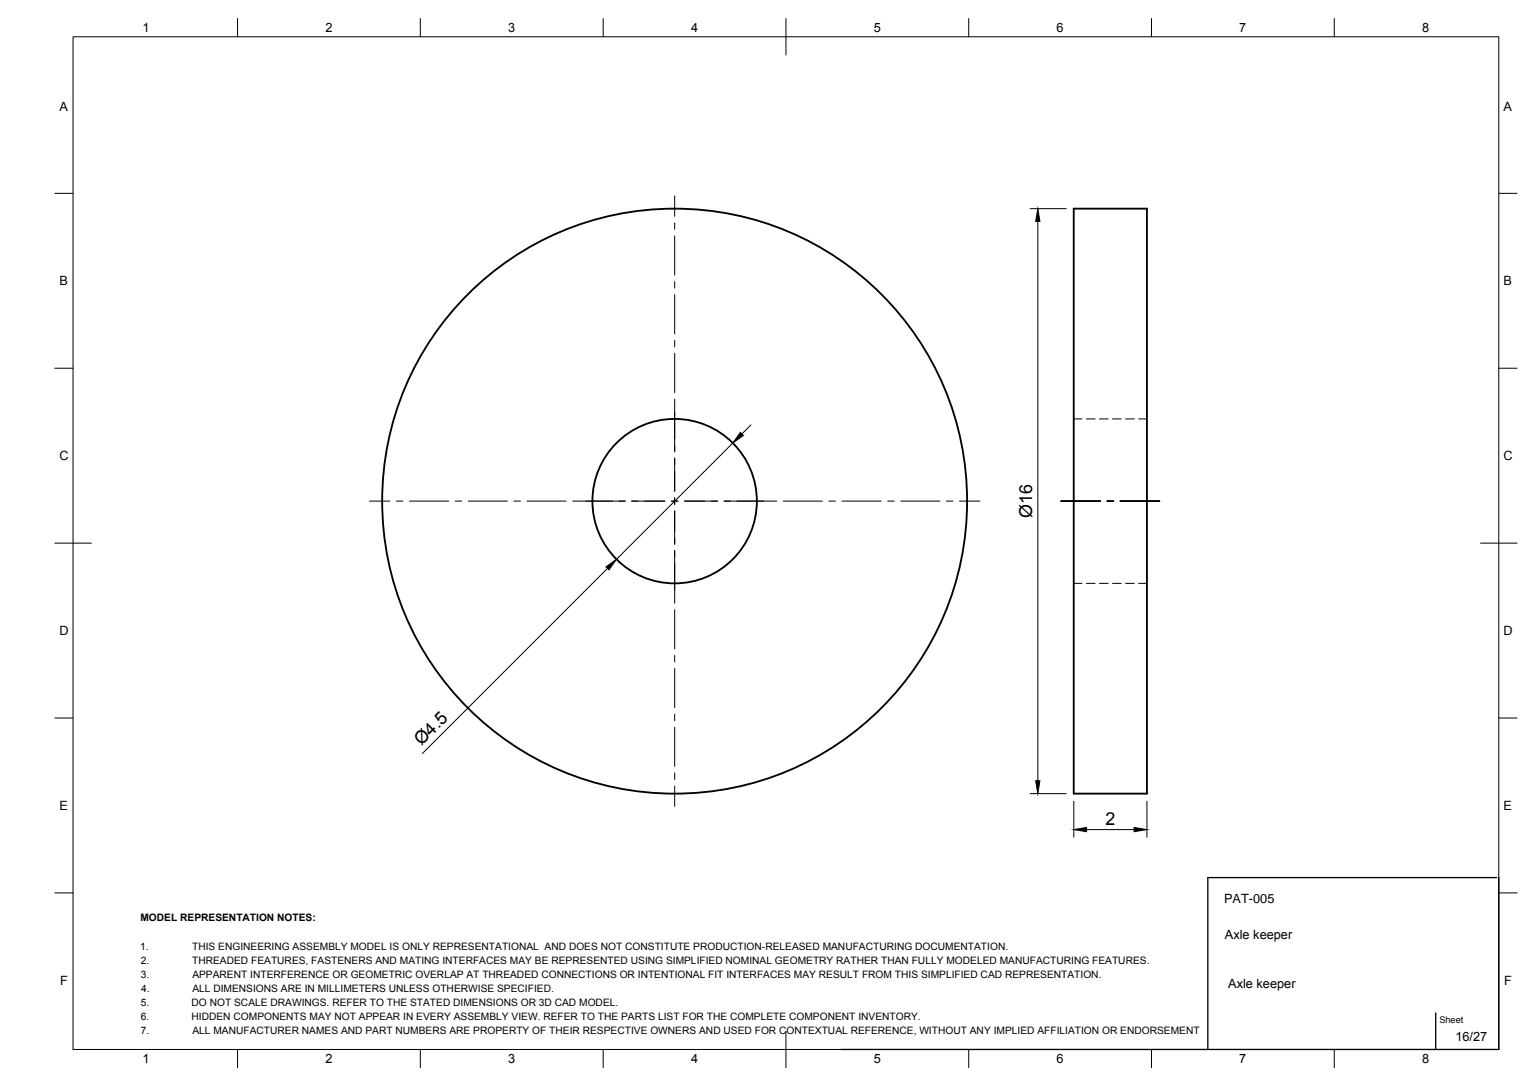
ISO-10303-21;
HEADER;
/* Generated by software containing ST-Developer
 * from STEP Tools, Inc. (www.steptools.com) 
 */

FILE_DESCRIPTION(
/* description */ ('Ball-race swivel caster'),
/* implementation_level */ '2;1');

FILE_NAME(
/* name */ 'Axle keeper.step',
/* time_stamp */ '2026-10-29T16:15:51-07:00',
/* author */ (''),
/* organization */ (''),
/* preprocessor_version */ 'ST-DEVELOPER v20.2',
/* originating_system */ 'Autodesk Translation Framework v15.17.0.0',
/* authorisation */ '');

FILE_SCHEMA (('AUTOMOTIVE_DESIGN { 1 0 10303 214 3 1 1 }'));
ENDSEC;

DATA;
#10=MECHANICAL_DESIGN_GEOMETRIC_PRESENTATION_REPRESENTATION('',(#318),#7816);
#269=SHAPE_REPRESENTATION_RELATIONSHIP('SRR','None',#7916,#289);
#289=ADVANCED_BREP_SHAPE_REPRESENTATION('',(#354),#7805);
#318=STYLED_ITEM('',(#8097),#354);
#354=MANIFOLD_SOLID_BREP('Body1',#3724);
#420=FACE_BOUND('',#916,.T.);
#421=FACE_BOUND('',#918,.T.);
#489=PLANE('',#4293);
#490=PLANE('',#4294);
#653=FACE_OUTER_BOUND('',#913,.T.);
#654=FACE_OUTER_BOUND('',#914,.T.);
#655=FACE_OUTER_BOUND('',#915,.T.);
#656=FACE_OUTER_BOUND('',#917,.T.);
#913=EDGE_LOOP('',(#3121,#3122,#3123,#3124));
#914=EDGE_LOOP('',(#3125,#3126,#3127,#3128));
#915=EDGE_LOOP('',(#3129));
#916=EDGE_LOOP('',(#3130));
#917=EDGE_LOOP('',(#3131));
#918=EDGE_LOOP('',(#3132));
#1119=LINE('',#7101,#1274);
#1120=LINE('',#7107,#1275);
#1274=VECTOR('',#5251,0.225);
#1275=VECTOR('',#5258,0.8);
#1493=CIRCLE('',#4288,0.225);
#1494=CIRCLE('',#4289,0.225);
#1495=CIRCLE('',#4291,0.8);
#1496=CIRCLE('',#4292,0.8);
#1827=VERTEX_POINT('',#7098);
#1828=VERTEX_POINT('',#7100);
#1829=VERTEX_POINT('',#7104);
#1830=VERTEX_POINT('',#7106);
#2280=EDGE_CURVE('',#1827,#1827,#1493,.T.);
#2281=EDGE_CURVE('',#1827,#1828,#1119,.T.);
#2282=EDGE_CURVE('',#1828,#1828,#1494,.T.);
#2283=EDGE_CURVE('',#1829,#1829,#1495,.T.);
#2284=EDGE_CURVE('',#1829,#1830,#1120,.T.);
#2285=EDGE_CURVE('',#1830,#1830,#1496,.T.);
#3121=ORIENTED_EDGE('',*,*,#2280,.F.);
#3122=ORIENTED_EDGE('',*,*,#2281,.T.);
#3123=ORIENTED_EDGE('',*,*,#2282,.T.);
#3124=ORIENTED_EDGE('',*,*,#2281,.F.);
#3125=ORIENTED_EDGE('',*,*,#2283,.F.);
#3126=ORIENTED_EDGE('',*,*,#2284,.T.);
#3127=ORIENTED_EDGE('',*,*,#2285,.T.);
#3128=ORIENTED_EDGE('',*,*,#2284,.F.);
#3129=ORIENTED_EDGE('',*,*,#2283,.T.);
#3130=ORIENTED_EDGE('',*,*,#2280,.T.);
#3131=ORIENTED_EDGE('',*,*,#2285,.F.);
#3132=ORIENTED_EDGE('',*,*,#2282,.F.);
#3473=CYLINDRICAL_SURFACE('',#4287,0.225);
#3474=CYLINDRICAL_SURFACE('',#4290,0.8);
#3624=ADVANCED_FACE('',(#653),#3473,.F.);
#3625=ADVANCED_FACE('',(#654),#3474,.T.);
#3626=ADVANCED_FACE('',(#655,#420),#489,.T.);
#3627=ADVANCED_FACE('',(#656,#421),#490,.F.);
#3724=CLOSED_SHELL('',(#3624,#3625,#3626,#3627));
#4286=AXIS2_PLACEMENT_3D('',#7096,#5245,#5246);
#4287=AXIS2_PLACEMENT_3D('',#7097,#5247,#5248);
#4288=AXIS2_PLACEMENT_3D('',#7099,#5249,#5250);
#4289=AXIS2_PLACEMENT_3D('',#7102,#5252,#5253);
#4290=AXIS2_PLACEMENT_3D('',#7103,#5254,#5255);
#4291=AXIS2_PLACEMENT_3D('',#7105,#5256,#5257);
#4292=AXIS2_PLACEMENT_3D('',#7108,#5259,#5260);
#4293=AXIS2_PLACEMENT_3D('',#7109,#5261,#5262);
#4294=AXIS2_PLACEMENT_3D('',#7110,#5263,#5264);
#5245=DIRECTION('axis',(0.,0.,1.));
#5246=DIRECTION('refdir',(1.,0.,0.));
#5247=DIRECTION('center_axis',(0.,1.,0.));
#5248=DIRECTION('ref_axis',(1.,0.,0.));
#5249=DIRECTION('center_axis',(0.,-1.,0.));
#5250=DIRECTION('ref_axis',(1.,0.,0.));
#5251=DIRECTION('',(0.,-1.,0.));
#5252=DIRECTION('center_axis',(0.,-1.,0.));
#5253=DIRECTION('ref_axis',(1.,0.,0.));
#5254=DIRECTION('center_axis',(0.,1.,0.));
#5255=DIRECTION('ref_axis',(1.,0.,0.));
#5256=DIRECTION('center_axis',(0.,1.,0.));
#5257=DIRECTION('ref_axis',(1.,0.,0.));
#5258=DIRECTION('',(0.,-1.,0.));
#5259=DIRECTION('center_axis',(0.,1.,0.));
#5260=DIRECTION('ref_axis',(1.,0.,0.));
#5261=DIRECTION('center_axis',(0.,1.,0.));
#5262=DIRECTION('ref_axis',(1.,0.,0.));
#5263=DIRECTION('center_axis',(0.,1.,0.));
#5264=DIRECTION('ref_axis',(1.,0.,0.));
#7096=CARTESIAN_POINT('',(0.,0.,0.));
#7097=CARTESIAN_POINT('Origin',(0.,2.2,4.));
#7098=CARTESIAN_POINT('',(-0.225,2.4,4.));
#7099=CARTESIAN_POINT('Origin',(0.,2.4,4.));
#7100=CARTESIAN_POINT('',(-0.225,2.2,4.));
#7101=CARTESIAN_POINT('',(-0.225,2.2,4.));
#7102=CARTESIAN_POINT('Origin',(0.,2.2,4.));
#7103=CARTESIAN_POINT('Origin',(0.,2.2,4.));
#7104=CARTESIAN_POINT('',(-0.8,2.4,4.));
#7105=CARTESIAN_POINT('Origin',(0.,2.4,4.));
#7106=CARTESIAN_POINT('',(-0.8,2.2,4.));
#7107=CARTESIAN_POINT('',(-0.8,2.2,4.));
#7108=CARTESIAN_POINT('Origin',(0.,2.2,4.));
#7109=CARTESIAN_POINT('Origin',(0.,2.4,4.));
#7110=CARTESIAN_POINT('Origin',(0.,2.2,4.));
#7778=UNCERTAINTY_MEASURE_WITH_UNIT(LENGTH_MEASURE(0.001),#7817,
'DISTANCE_ACCURACY_VALUE',
'Maximum model space distance between geometric entities at asserted c
onnectivities');
#7789=UNCERTAINTY_MEASURE_WITH_UNIT(LENGTH_MEASURE(0.001),#7817,
'DISTANCE_ACCURACY_VALUE',
'Maximum model space distance between geometric entities at asserted c
onnectivities');
#7805=(
GEOMETRIC_REPRESENTATION_CONTEXT(3)
GLOBAL_UNCERTAINTY_ASSIGNED_CONTEXT((#7778))
GLOBAL_UNIT_ASSIGNED_CONTEXT((#7817,#7819,#7820))
REPRESENTATION_CONTEXT('','3D')
);
#7816=(
GEOMETRIC_REPRESENTATION_CONTEXT(3)
GLOBAL_UNCERTAINTY_ASSIGNED_CONTEXT((#7789))
GLOBAL_UNIT_ASSIGNED_CONTEXT((#7817,#7819,#7820))
REPRESENTATION_CONTEXT('','3D')
);
#7817=(
LENGTH_UNIT()
NAMED_UNIT(*)
SI_UNIT(.CENTI.,.METRE.)
);
#7819=(
NAMED_UNIT(*)
PLANE_ANGLE_UNIT()
SI_UNIT($,.RADIAN.)
);
#7820=(
NAMED_UNIT(*)
SI_UNIT($,.STERADIAN.)
SOLID_ANGLE_UNIT()
);
#7836=SHAPE_DEFINITION_REPRESENTATION(#7870,#7916);
#7870=PRODUCT_DEFINITION_SHAPE('',$,#7943);
#7916=SHAPE_REPRESENTATION('',(#4286),#7805);
#7927=PRODUCT_DEFINITION_CONTEXT('part definition',#8007,'design');
#7943=PRODUCT_DEFINITION('Axle keeper','Axle keeper',#7969,#7927);
#7969=PRODUCT_DEFINITION_FORMATION('',$,#8024);
#8007=APPLICATION_CONTEXT(
'Core Data for Automotive Mechanical Design Process');
#8008=PRODUCT_CONTEXT('part definition',#8007,'mechanical');
#8024=PRODUCT('Axle keeper','Axle keeper','Axle keeper',(#8008));
#8091=COLOUR_RGB('Grey',0.48,0.52,0.57);
#8092=FILL_AREA_STYLE_COLOUR('',#8091);
#8093=FILL_AREA_STYLE('',(#8092));
#8094=SURFACE_STYLE_FILL_AREA(#8093);
#8095=SURFACE_SIDE_STYLE('',(#8094));
#8096=SURFACE_STYLE_USAGE(.BOTH.,#8095);
#8097=PRESENTATION_STYLE_ASSIGNMENT((#8096));
ENDSEC;
END-ISO-10303-21;
